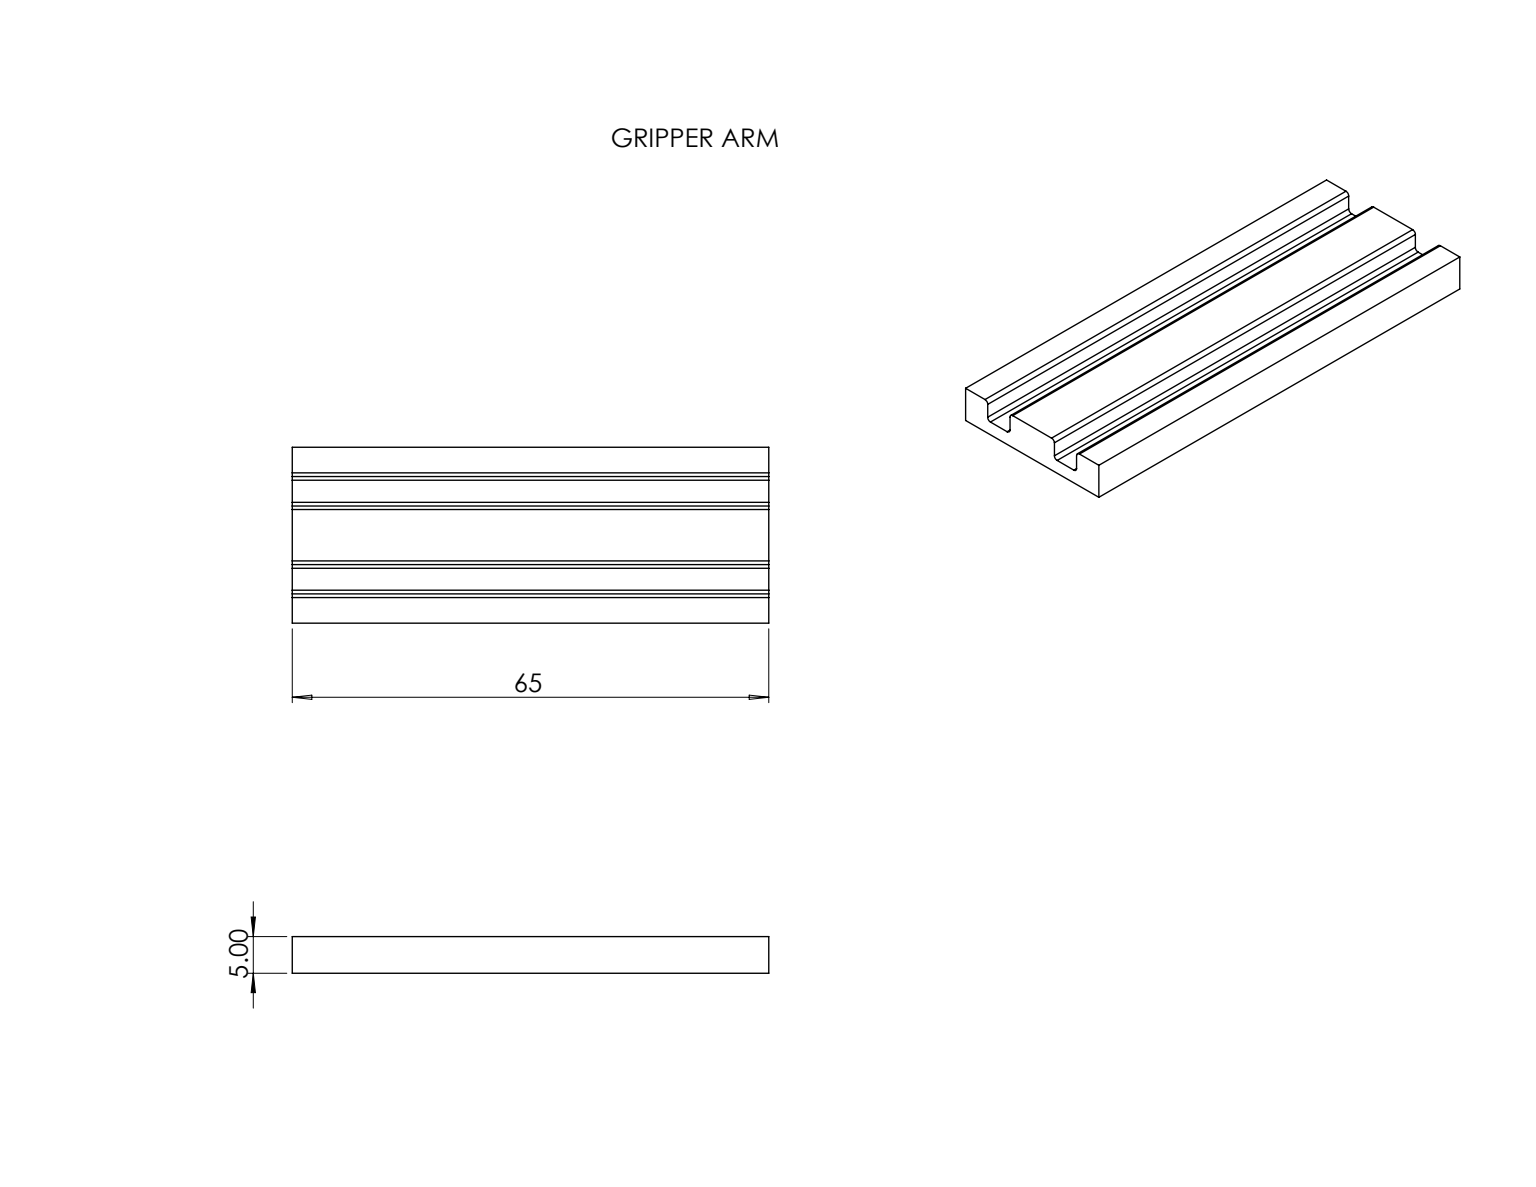
ISO-10303-21;
HEADER;
FILE_DESCRIPTION (('STEP AP214'),
    '1' );
FILE_NAME ('Gripper Arm.step',
    '2026-10-07T17:53:07',
    ( '' ),
    ( '' ),
    'SwSTEP 2.0',
    'SolidWorks 2025',
    '' );
FILE_SCHEMA (( 'AUTOMOTIVE_DESIGN' ));
ENDSEC;

DATA;
#37=( GEOMETRIC_REPRESENTATION_CONTEXT ( 3 ) GLOBAL_UNCERTAINTY_ASSIGNED_CONTEXT ( ( #1666 ) ) GLOBAL_UNIT_ASSIGNED_CONTEXT ( ( #5163, #1674, #7109 ) ) REPRESENTATION_CONTEXT ( 'NONE', 'WORKASPACE' ) );
#80=EDGE_CURVE ( 'NONE', #9144, #4985, #2152, .T. ) ;
#98=DIRECTION ( 'NONE',  ( 0.000000000000000000, 0.000000000000000000, 1.000000000000000000 ) ) ;
#126=EDGE_CURVE ( 'NONE', #1534, #5295, #6389, .T. ) ;
#133=DIRECTION ( 'NONE',  ( 0.000000000000000000, 0.000000000000000000, 1.000000000000000000 ) ) ;
#157=SHAPE_DEFINITION_REPRESENTATION ( #3699, #5502 ) ;
#159=VERTEX_POINT ( 'NONE', #3135 ) ;
#161=EDGE_CURVE ( 'NONE', #11468, #4985, #9362, .T. ) ;
#166=VECTOR ( 'NONE', #7008, 1000.000000000000000 ) ;
#169=CARTESIAN_POINT ( 'NONE',  ( 3.500000000000001776, 2.000000000000000000, 0.000000000000000000 ) ) ;
#177=VECTOR ( 'NONE', #8514, 1000.000000000000000 ) ;
#257=CYLINDRICAL_SURFACE ( 'NONE', #13000, 0.5000000000000004441 ) ;
#264=CARTESIAN_POINT ( 'NONE',  ( -3.499999999999998224, 2.499999999999999556, 0.000000000000000000 ) ) ;
#274=DIRECTION ( 'NONE',  ( 0.000000000000000000, 1.000000000000000000, 0.000000000000000000 ) ) ;
#275=FACE_OUTER_BOUND ( 'NONE', #13534, .T. ) ;
#280=VECTOR ( 'NONE', #607, 1000.000000000000000 ) ;
#294=DIRECTION ( 'NONE',  ( 0.000000000000000000, 0.000000000000000000, 1.000000000000000000 ) ) ;
#317=ORIENTED_EDGE ( 'NONE', *, *, #5380, .F. ) ;
#339=DIRECTION ( 'NONE',  ( -0.000000000000000000, -0.000000000000000000, -1.000000000000000000 ) ) ;
#366=ORIENTED_EDGE ( 'NONE', *, *, #1120, .F. ) ;
#378=LINE ( 'NONE', #13236, #10194 ) ;
#379=ORIENTED_EDGE ( 'NONE', *, *, #12753, .T. ) ;
#391=ORIENTED_EDGE ( 'NONE', *, *, #1074, .T. ) ;
#401=LINE ( 'NONE', #12069, #13543 ) ;
#408=DIRECTION ( 'NONE',  ( -1.239088197126292296E-16, 1.000000000000000000, 0.000000000000000000 ) ) ;
#414=EDGE_CURVE ( 'NONE', #159, #13667, #776, .T. ) ;
#426=CARTESIAN_POINT ( 'NONE',  ( -7.499999999999996447, -0.5000000000000019984, 0.000000000000000000 ) ) ;
#427=PLANE ( 'NONE',  #8021 ) ;
#431=ORIENTED_EDGE ( 'NONE', *, *, #1519, .T. ) ;
#490=EDGE_CURVE ( 'NONE', #10813, #8384, #10834, .T. ) ;
#544=EDGE_CURVE ( 'NONE', #2553, #8162, #1184, .T. ) ;
#571=ORIENTED_EDGE ( 'NONE', *, *, #161, .T. ) ;
#607=DIRECTION ( 'NONE',  ( -1.000000000000000000, -1.239088197126292296E-16, -0.000000000000000000 ) ) ;
#627=DIRECTION ( 'NONE',  ( -0.000000000000000000, -0.000000000000000000, -1.000000000000000000 ) ) ;
#631=ORIENTED_EDGE ( 'NONE', *, *, #12993, .T. ) ;
#646=CIRCLE ( 'NONE', #2677, 0.5000000000000004441 ) ;
#654=CARTESIAN_POINT ( 'NONE',  ( 4.500000000000002665, -0.5000000000000005551, 0.000000000000000000 ) ) ;
#657=LINE ( 'NONE', #12469, #5078 ) ;
#683=VECTOR ( 'NONE', #6615, 1000.000000000000000 ) ;
#685=ORIENTED_EDGE ( 'NONE', *, *, #926, .F. ) ;
#687=DIRECTION ( 'NONE',  ( 1.000000000000000000, 0.000000000000000000, 0.000000000000000000 ) ) ;
#694=FACE_OUTER_BOUND ( 'NONE', #1462, .T. ) ;
#736=EDGE_CURVE ( 'NONE', #4755, #1534, #2879, .T. ) ;
#748=DIRECTION ( 'NONE',  ( -0.000000000000000000, -0.000000000000000000, -1.000000000000000000 ) ) ;
#776=LINE ( 'NONE', #13553, #11837 ) ;
#789=EDGE_CURVE ( 'NONE', #2553, #2266, #4127, .T. ) ;
#797=DIRECTION ( 'NONE',  ( 0.000000000000000000, 0.000000000000000000, 1.000000000000000000 ) ) ;
#825=SURFACE_SIDE_STYLE ('',( #2881 ) ) ;
#870=CARTESIAN_POINT ( 'NONE',  ( 3.500000000000001776, 2.000000000000000000, -65.00000000000000000 ) ) ;
#886=FACE_OUTER_BOUND ( 'NONE', #3660, .T. ) ;
#891=ADVANCED_FACE ( 'NONE', ( #3224 ), #10819, .T. ) ;
#901=DIRECTION ( 'NONE',  ( 0.000000000000000000, 0.000000000000000000, 1.000000000000000000 ) ) ;
#904=EDGE_CURVE ( 'NONE', #3647, #3770, #5487, .T. ) ;
#905=AXIS2_PLACEMENT_3D ( 'NONE', #10351, #13424, #6008 ) ;
#926=EDGE_CURVE ( 'NONE', #10303, #13667, #5427, .T. ) ;
#928=EDGE_CURVE ( 'NONE', #1230, #2349, #8492, .T. ) ;
#934=ADVANCED_FACE ( 'NONE', ( #275 ), #5359, .T. ) ;
#992=CARTESIAN_POINT ( 'NONE',  ( -7.499999999999996447, -1.762812401309176307E-15, -65.00000000000000000 ) ) ;
#1016=DIRECTION ( 'NONE',  ( 1.000000000000000000, 0.000000000000000000, 0.000000000000000000 ) ) ;
#1074=EDGE_CURVE ( 'NONE', #2266, #4291, #7792, .T. ) ;
#1075=( GEOMETRIC_REPRESENTATION_CONTEXT ( 3 ) GLOBAL_UNCERTAINTY_ASSIGNED_CONTEXT ( ( #1813 ) ) GLOBAL_UNIT_ASSIGNED_CONTEXT ( ( #10879, #7487, #2162 ) ) REPRESENTATION_CONTEXT ( 'NONE', 'WORKASPACE' ) );
#1077=ORIENTED_EDGE ( 'NONE', *, *, #9933, .F. ) ;
#1098=DIRECTION ( 'NONE',  ( -1.000000000000000000, 5.059610138265691632E-16, 0.000000000000000000 ) ) ;
#1120=EDGE_CURVE ( 'NONE', #8521, #2257, #4929, .T. ) ;
#1162=ORIENTED_EDGE ( 'NONE', *, *, #6210, .T. ) ;
#1167=EDGE_CURVE ( 'NONE', #10572, #8384, #2508, .T. ) ;
#1184=LINE ( 'NONE', #9716, #3596 ) ;
#1192=LINE ( 'NONE', #12999, #11798 ) ;
#1196=ORIENTED_EDGE ( 'NONE', *, *, #10990, .T. ) ;
#1222=CARTESIAN_POINT ( 'NONE',  ( -8.500000000000000000, 2.499999999999999556, -65.00000000000000000 ) ) ;
#1230=VERTEX_POINT ( 'NONE', #9272 ) ;
#1245=ORIENTED_EDGE ( 'NONE', *, *, #8673, .T. ) ;
#1246=VECTOR ( 'NONE', #11216, 1000.000000000000000 ) ;
#1258=ORIENTED_EDGE ( 'NONE', *, *, #10990, .F. ) ;
#1259=ORIENTED_EDGE ( 'NONE', *, *, #7216, .F. ) ;
#1303=FACE_OUTER_BOUND ( 'NONE', #3883, .T. ) ;
#1373=CARTESIAN_POINT ( 'NONE',  ( 3.500000000000001776, 2.499999999999999556, 0.000000000000000000 ) ) ;
#1380=DIRECTION ( 'NONE',  ( -1.000000000000000000, -2.529805069132845816E-16, 0.000000000000000000 ) ) ;
#1385=CARTESIAN_POINT ( 'NONE',  ( 7.500000000000000000, -0.5000000000000017764, -65.00000000000000000 ) ) ;
#1407=EDGE_CURVE ( 'NONE', #8384, #9884, #13503, .T. ) ;
#1437=PLANE ( 'NONE',  #8954 ) ;
#1462=EDGE_LOOP ( 'NONE', ( #7418, #7086, #12382, #7454 ) ) ;
#1476=ORIENTED_EDGE ( 'NONE', *, *, #13544, .T. ) ;
#1493=EDGE_LOOP ( 'NONE', ( #9757, #11508, #6256, #13606 ) ) ;
#1519=EDGE_CURVE ( 'NONE', #5154, #11963, #6379, .T. ) ;
#1534=VERTEX_POINT ( 'NONE', #11903 ) ;
#1608=COLOUR_RGB ( '', 0.08235294, 0.09019608, 0.10196078) ;
#1613=DIRECTION ( 'NONE',  ( 1.000000000000000000, 0.000000000000000000, -0.000000000000000000 ) ) ;
#1620=ORIENTED_EDGE ( 'NONE', *, *, #9892, .T. ) ;
#1648=EDGE_CURVE ( 'NONE', #4985, #10572, #10929, .T. ) ;
#1649=EDGE_LOOP ( 'NONE', ( #12050, #2259, #5190, #4837 ) ) ;
#1658=ORIENTED_EDGE ( 'NONE', *, *, #1074, .F. ) ;
#1660=LINE ( 'NONE', #7289, #5099 ) ;
#1666=UNCERTAINTY_MEASURE_WITH_UNIT (LENGTH_MEASURE( 1.000000000000000082E-05 ), #5163, 'distance_accuracy_value', 'NONE');
#1671=ORIENTED_EDGE ( 'NONE', *, *, #1519, .F. ) ;
#1674=( NAMED_UNIT ( * ) PLANE_ANGLE_UNIT ( ) SI_UNIT ( $, .RADIAN. ) );
#1706=DIRECTION ( 'NONE',  ( 0.000000000000000000, 0.000000000000000000, 1.000000000000000000 ) ) ;
#1719=ORIENTED_EDGE ( 'NONE', *, *, #11656, .T. ) ;
#1745=AXIS2_PLACEMENT_3D ( 'NONE', #12207, #274, #3424 ) ;
#1764=CARTESIAN_POINT ( 'NONE',  ( 12.00000000000000000, -2.499999999999999556, -65.00000000000000000 ) ) ;
#1796=CARTESIAN_POINT ( 'NONE',  ( 7.500000000000000000, -0.5000000000000017764, 0.000000000000000000 ) ) ;
#1813=UNCERTAINTY_MEASURE_WITH_UNIT (LENGTH_MEASURE( 1.000000000000000082E-05 ), #10879, 'distance_accuracy_value', 'NONE');
#1815=AXIS2_PLACEMENT_3D ( 'NONE', #2245, #11724, #9640 ) ;
#1823=DIRECTION ( 'NONE',  ( 0.000000000000000000, 0.000000000000000000, 1.000000000000000000 ) ) ;
#1859=CARTESIAN_POINT ( 'NONE',  ( -4.499999999999999112, -1.301042606982605321E-15, -65.00000000000000000 ) ) ;
#1900=ORIENTED_EDGE ( 'NONE', *, *, #12612, .F. ) ;
#1914=ORIENTED_EDGE ( 'NONE', *, *, #5344, .T. ) ;
#1917=EDGE_CURVE ( 'NONE', #3017, #10813, #3374, .T. ) ;
#1919=AXIS2_PLACEMENT_3D ( 'NONE', #10965, #5557, #1380 ) ;
#1940=LINE ( 'NONE', #6111, #280 ) ;
#1965=ADVANCED_FACE ( 'NONE', ( #10130 ), #10060, .T. ) ;
#1983=DIRECTION ( 'NONE',  ( 0.000000000000000000, 0.000000000000000000, 1.000000000000000000 ) ) ;
#1992=VECTOR ( 'NONE', #10685, 1000.000000000000000 ) ;
#1999=ORIENTED_EDGE ( 'NONE', *, *, #9250, .F. ) ;
#2000=AXIS2_PLACEMENT_3D ( 'NONE', #6057, #11507, #10460 ) ;
#2018=AXIS2_PLACEMENT_3D ( 'NONE', #10654, #10728, #1016 ) ;
#2048=VECTOR ( 'NONE', #8009, 1000.000000000000000 ) ;
#2065=VECTOR ( 'NONE', #4779, 1000.000000000000000 ) ;
#2114=ADVANCED_FACE ( 'NONE', ( #886 ), #7167, .T. ) ;
#2151=CARTESIAN_POINT ( 'NONE',  ( 4.500000000000002665, -0.5000000000000005551, -65.00000000000000000 ) ) ;
#2152=LINE ( 'NONE', #12953, #13752 ) ;
#2153=LINE ( 'NONE', #4239, #9391 ) ;
#2160=DIRECTION ( 'NONE',  ( 0.000000000000000000, 1.000000000000000000, 0.000000000000000000 ) ) ;
#2162=( NAMED_UNIT ( * ) SI_UNIT ( $, .STERADIAN. ) SOLID_ANGLE_UNIT ( ) );
#2168=ORIENTED_EDGE ( 'NONE', *, *, #126, .T. ) ;
#2172=DIRECTION ( 'NONE',  ( 1.000000000000000000, 0.000000000000000000, 0.000000000000000000 ) ) ;
#2205=CARTESIAN_POINT ( 'NONE',  ( 8.500000000000003553, 2.500000000000000000, 0.000000000000000000 ) ) ;
#2239=ORIENTED_EDGE ( 'NONE', *, *, #7229, .F. ) ;
#2245=CARTESIAN_POINT ( 'NONE',  ( 8.500000000000001776, 2.000000000000000000, -65.00000000000000000 ) ) ;
#2257=VERTEX_POINT ( 'NONE', #10663 ) ;
#2259=ORIENTED_EDGE ( 'NONE', *, *, #544, .F. ) ;
#2266=VERTEX_POINT ( 'NONE', #6674 ) ;
#2306=EDGE_CURVE ( 'NONE', #4291, #159, #7705, .T. ) ;
#2347=VERTEX_POINT ( 'NONE', #1373 ) ;
#2349=VERTEX_POINT ( 'NONE', #1222 ) ;
#2367=VERTEX_POINT ( 'NONE', #7563 ) ;
#2380=VERTEX_POINT ( 'NONE', #4381 ) ;
#2389=CARTESIAN_POINT ( 'NONE',  ( -3.499999999999998224, 2.499999999999999556, -65.00000000000000000 ) ) ;
#2409=ADVANCED_FACE ( 'NONE', ( #5828 ), #1437, .T. ) ;
#2462=VECTOR ( 'NONE', #11651, 1000.000000000000000 ) ;
#2466=LINE ( 'NONE', #9005, #10134 ) ;
#2497=DIRECTION ( 'NONE',  ( -0.000000000000000000, 1.000000000000000000, -0.000000000000000000 ) ) ;
#2508=CIRCLE ( 'NONE', #6274, 0.5000000000000004441 ) ;
#2511=CARTESIAN_POINT ( 'NONE',  ( -7.999999999999996447, -1.701580061351808733E-15, -65.00000000000000000 ) ) ;
#2540=ORIENTED_EDGE ( 'NONE', *, *, #4860, .F. ) ;
#2553=VERTEX_POINT ( 'NONE', #11356 ) ;
#2677=AXIS2_PLACEMENT_3D ( 'NONE', #10326, #748, #9275 ) ;
#2689=VECTOR ( 'NONE', #6333, 1000.000000000000000 ) ;
#2717=LINE ( 'NONE', #11284, #6753 ) ;
#2718=LINE ( 'NONE', #7210, #166 ) ;
#2741=CARTESIAN_POINT ( 'NONE',  ( 12.00000000000000000, 2.500000000000000000, 0.000000000000000000 ) ) ;
#2848=ORIENTED_EDGE ( 'NONE', *, *, #6277, .F. ) ;
#2852=DIRECTION ( 'NONE',  ( 0.000000000000000000, 0.000000000000000000, 1.000000000000000000 ) ) ;
#2854=DIRECTION ( 'NONE',  ( 0.000000000000000000, 0.000000000000000000, 1.000000000000000000 ) ) ;
#2879=LINE ( 'NONE', #13538, #11401 ) ;
#2881=SURFACE_STYLE_FILL_AREA ( #13409 ) ;
#2904=CYLINDRICAL_SURFACE ( 'NONE', #9563, 0.5000000000000004441 ) ;
#2965=EDGE_CURVE ( 'NONE', #13584, #12422, #13356, .T. ) ;
#2983=CARTESIAN_POINT ( 'NONE',  ( 8.000000000000000000, -1.762812401309176307E-15, -65.00000000000000000 ) ) ;
#3017=VERTEX_POINT ( 'NONE', #2983 ) ;
#3031=CYLINDRICAL_SURFACE ( 'NONE', #5960, 0.4999999999999991673 ) ;
#3071=CARTESIAN_POINT ( 'NONE',  ( 7.500000000000000000, -1.762812401309176307E-15, 0.000000000000000000 ) ) ;
#3082=FACE_OUTER_BOUND ( 'NONE', #12101, .T. ) ;
#3085=CARTESIAN_POINT ( 'NONE',  ( -12.00000000000000000, -2.500000000000000444, -65.00000000000000000 ) ) ;
#3099=CIRCLE ( 'NONE', #8884, 0.4999999999999991673 ) ;
#3131=EDGE_CURVE ( 'NONE', #11544, #11152, #4409, .T. ) ;
#3135=CARTESIAN_POINT ( 'NONE',  ( 12.00000000000000000, 2.500000000000000000, -65.00000000000000000 ) ) ;
#3142=CARTESIAN_POINT ( 'NONE',  ( 4.000000000000001776, 2.000000000000000000, -65.00000000000000000 ) ) ;
#3216=ORIENTED_EDGE ( 'NONE', *, *, #6210, .F. ) ;
#3224=FACE_OUTER_BOUND ( 'NONE', #4359, .T. ) ;
#3259=ADVANCED_FACE ( 'NONE', ( #6715 ), #427, .T. ) ;
#3263=ADVANCED_FACE ( 'NONE', ( #6840 ), #9932, .T. ) ;
#3276=CARTESIAN_POINT ( 'NONE',  ( -12.00000000000000000, 2.500000000000000000, 0.000000000000000000 ) ) ;
#3336=DIRECTION ( 'NONE',  ( 0.000000000000000000, -1.000000000000000000, 0.000000000000000000 ) ) ;
#3343=EDGE_LOOP ( 'NONE', ( #5355, #571, #8847, #13069, #9284, #8231, #13676, #5582, #12581, #8099, #2168, #9530, #11277, #5885, #6832, #13165, #1162, #8173, #631, #10642 ) ) ;
#3344=ORIENTED_EDGE ( 'NONE', *, *, #8167, .F. ) ;
#3350=VECTOR ( 'NONE', #13795, 1000.000000000000000 ) ;
#3374=CIRCLE ( 'NONE', #10066, 0.5000000000000004441 ) ;
#3407=DIRECTION ( 'NONE',  ( 0.000000000000000000, 0.000000000000000000, 1.000000000000000000 ) ) ;
#3412=CARTESIAN_POINT ( 'NONE',  ( 12.00000000000000000, -2.499999999999999556, -65.00000000000000000 ) ) ;
#3417=ORIENTED_EDGE ( 'NONE', *, *, #904, .F. ) ;
#3424=DIRECTION ( 'NONE',  ( 0.000000000000000000, -0.000000000000000000, 1.000000000000000000 ) ) ;
#3455=EDGE_CURVE ( 'NONE', #11963, #3647, #4031, .T. ) ;
#3464=ORIENTED_EDGE ( 'NONE', *, *, #12753, .F. ) ;
#3488=DIRECTION ( 'NONE',  ( -1.000000000000000000, 0.000000000000000000, 0.000000000000000000 ) ) ;
#3516=ORIENTED_EDGE ( 'NONE', *, *, #12993, .F. ) ;
#3517=VECTOR ( 'NONE', #7581, 1000.000000000000000 ) ;
#3559=CARTESIAN_POINT ( 'NONE',  ( -12.00000000000000000, -2.500000000000000444, 0.000000000000000000 ) ) ;
#3588=ORIENTED_EDGE ( 'NONE', *, *, #8167, .T. ) ;
#3591=ORIENTED_EDGE ( 'NONE', *, *, #1120, .T. ) ;
#3592=EDGE_CURVE ( 'NONE', #3770, #4357, #4258, .T. ) ;
#3596=VECTOR ( 'NONE', #4403, 1000.000000000000000 ) ;
#3612=CARTESIAN_POINT ( 'NONE',  ( 8.000000000000001776, 2.000000000000000000, -65.00000000000000000 ) ) ;
#3627=VERTEX_POINT ( 'NONE', #3559 ) ;
#3647=VERTEX_POINT ( 'NONE', #12974 ) ;
#3660=EDGE_LOOP ( 'NONE', ( #9021, #12465, #5916, #10909 ) ) ;
#3664=CARTESIAN_POINT ( 'NONE',  ( 3.500000000000001776, 2.499999999999999556, -65.00000000000000000 ) ) ;
#3687=CARTESIAN_POINT ( 'NONE',  ( -8.499999999999998224, 2.000000000000000000, 0.000000000000000000 ) ) ;
#3697=CARTESIAN_POINT ( 'NONE',  ( -12.00000000000000000, -2.500000000000000444, -65.00000000000000000 ) ) ;
#3699=PRODUCT_DEFINITION_SHAPE ( 'NONE', 'NONE',  #10061 ) ;
#3744=PLANE ( 'NONE',  #4196 ) ;
#3753=CARTESIAN_POINT ( 'NONE',  ( -12.00000000000000000, 2.500000000000000000, 0.000000000000000000 ) ) ;
#3754=DIRECTION ( 'NONE',  ( 1.000000000000000000, 0.000000000000000000, 0.000000000000000000 ) ) ;
#3770=VERTEX_POINT ( 'NONE', #6047 ) ;
#3843=DIRECTION ( 'NONE',  ( -1.000000000000000000, 0.000000000000000000, 0.000000000000000000 ) ) ;
#3883=EDGE_LOOP ( 'NONE', ( #10092, #9235, #13516, #431 ) ) ;
#3888=CYLINDRICAL_SURFACE ( 'NONE', #9321, 0.5000000000000004441 ) ;
#3948=EDGE_CURVE ( 'NONE', #6401, #1534, #10955, .T. ) ;
#3970=EDGE_CURVE ( 'NONE', #8162, #3627, #2153, .T. ) ;
#3977=DIRECTION ( 'NONE',  ( 1.000000000000000000, 8.673617379884027583E-16, -0.000000000000000000 ) ) ;
#3998=VERTEX_POINT ( 'NONE', #10589 ) ;
#4031=CIRCLE ( 'NONE', #10940, 0.5000000000000004441 ) ;
#4080=CARTESIAN_POINT ( 'NONE',  ( -12.00000000000000000, 2.500000000000000000, -65.00000000000000000 ) ) ;
#4082=ORIENTED_EDGE ( 'NONE', *, *, #13544, .F. ) ;
#4088=ORIENTED_EDGE ( 'NONE', *, *, #6277, .T. ) ;
#4103=ORIENTED_EDGE ( 'NONE', *, *, #126, .F. ) ;
#4127=LINE ( 'NONE', #3085, #5364 ) ;
#4188=EDGE_LOOP ( 'NONE', ( #7507, #12754, #7359, #1914 ) ) ;
#4196=AXIS2_PLACEMENT_3D ( 'NONE', #7994, #6032, #8071 ) ;
#4239=CARTESIAN_POINT ( 'NONE',  ( -12.00000000000000000, -2.500000000000000444, 0.000000000000000000 ) ) ;
#4258=CIRCLE ( 'NONE', #13615, 0.5000000000000004441 ) ;
#4273=AXIS2_PLACEMENT_3D ( 'NONE', #10752, #8789, #2172 ) ;
#4284=CARTESIAN_POINT ( 'NONE',  ( 7.500000000000000000, -0.5000000000000017764, -65.00000000000000000 ) ) ;
#4289=VECTOR ( 'NONE', #4600, 1000.000000000000000 ) ;
#4291=VERTEX_POINT ( 'NONE', #1764 ) ;
#4301=AXIS2_PLACEMENT_3D ( 'NONE', #13028, #8910, #12053 ) ;
#4308=ADVANCED_FACE ( 'NONE', ( #4909 ), #9170, .T. ) ;
#4349=LINE ( 'NONE', #4284, #12699 ) ;
#4357=VERTEX_POINT ( 'NONE', #8454 ) ;
#4359=EDGE_LOOP ( 'NONE', ( #11012, #3344, #9662, #9926 ) ) ;
#4381=CARTESIAN_POINT ( 'NONE',  ( 4.000000000000001776, 2.000000000000000000, -65.00000000000000000 ) ) ;
#4403=DIRECTION ( 'NONE',  ( 0.000000000000000000, 0.000000000000000000, 1.000000000000000000 ) ) ;
#4409=LINE ( 'NONE', #10699, #5553 ) ;
#4446=DIRECTION ( 'NONE',  ( 1.000000000000000000, 0.000000000000000000, 0.000000000000000000 ) ) ;
#4537=FACE_OUTER_BOUND ( 'NONE', #9878, .T. ) ;
#4538=CARTESIAN_POINT ( 'NONE',  ( -7.999999999999998224, 2.000000000000000000, 0.000000000000000000 ) ) ;
#4554=DIRECTION ( 'NONE',  ( -0.000000000000000000, 0.000000000000000000, -1.000000000000000000 ) ) ;
#4556=CARTESIAN_POINT ( 'NONE',  ( -12.00000000000000000, -2.500000000000000444, -65.00000000000000000 ) ) ;
#4577=MANIFOLD_SOLID_BREP ( 'Boss-Extrude1', #5904 ) ;
#4600=DIRECTION ( 'NONE',  ( 0.000000000000000000, 0.000000000000000000, 1.000000000000000000 ) ) ;
#4658=DIRECTION ( 'NONE',  ( 1.000000000000000000, 3.614007241618347908E-17, 0.000000000000000000 ) ) ;
#4672=DIRECTION ( 'NONE',  ( -1.000000000000000000, -0.000000000000000000, -0.000000000000000000 ) ) ;
#4673=PLANE ( 'NONE',  #5961 ) ;
#4686=ORIENTED_EDGE ( 'NONE', *, *, #3131, .F. ) ;
#4697=DIRECTION ( 'NONE',  ( 0.000000000000000000, 0.000000000000000000, 1.000000000000000000 ) ) ;
#4723=PLANE ( 'NONE',  #6385 ) ;
#4755=VERTEX_POINT ( 'NONE', #8931 ) ;
#4762=DIRECTION ( 'NONE',  ( 1.000000000000000000, 0.000000000000000000, -0.000000000000000000 ) ) ;
#4779=DIRECTION ( 'NONE',  ( -8.673617379884027583E-16, -1.000000000000000000, 0.000000000000000000 ) ) ;
#4801=CARTESIAN_POINT ( 'NONE',  ( -3.999999999999997335, 2.000000000000000000, -65.00000000000000000 ) ) ;
#4814=EDGE_CURVE ( 'NONE', #1230, #3770, #13047, .T. ) ;
#4837=ORIENTED_EDGE ( 'NONE', *, *, #7216, .T. ) ;
#4860=EDGE_CURVE ( 'NONE', #159, #3998, #1940, .T. ) ;
#4909=FACE_OUTER_BOUND ( 'NONE', #10314, .T. ) ;
#4919=AXIS2_PLACEMENT_3D ( 'NONE', #11709, #9684, #9611 ) ;
#4925=DIRECTION ( 'NONE',  ( -1.000000000000000000, -2.529805069132845816E-16, -0.000000000000000000 ) ) ;
#4929=CIRCLE ( 'NONE', #12736, 0.5000000000000004441 ) ;
#4944=CARTESIAN_POINT ( 'NONE',  ( 8.000000000000001776, 2.000000000000000000, 0.000000000000000000 ) ) ;
#4956=PLANE ( 'NONE',  #8585 ) ;
#4985=VERTEX_POINT ( 'NONE', #4944 ) ;
#4990=DIRECTION ( 'NONE',  ( -1.000000000000000000, 0.000000000000000000, 0.000000000000000000 ) ) ;
#5078=VECTOR ( 'NONE', #4925, 1000.000000000000000 ) ;
#5079=CIRCLE ( 'NONE', #6862, 0.5000000000000004441 ) ;
#5099=VECTOR ( 'NONE', #8088, 1000.000000000000000 ) ;
#5107=DIRECTION ( 'NONE',  ( 0.000000000000000000, 0.000000000000000000, 1.000000000000000000 ) ) ;
#5154=VERTEX_POINT ( 'NONE', #9833 ) ;
#5163=( LENGTH_UNIT ( ) NAMED_UNIT ( * ) SI_UNIT ( .MILLI., .METRE. ) );
#5181=EDGE_CURVE ( 'NONE', #8888, #2367, #12766, .T. ) ;
#5186=EDGE_CURVE ( 'NONE', #13667, #11468, #13095, .T. ) ;
#5190=ORIENTED_EDGE ( 'NONE', *, *, #789, .T. ) ;
#5204=ORIENTED_EDGE ( 'NONE', *, *, #789, .F. ) ;
#5229=ADVANCED_FACE ( 'NONE', ( #8834 ), #257, .F. ) ;
#5290=CARTESIAN_POINT ( 'NONE',  ( -3.999999999999998224, -1.301042606982605321E-15, -65.00000000000000000 ) ) ;
#5295=VERTEX_POINT ( 'NONE', #5824 ) ;
#5302=CARTESIAN_POINT ( 'NONE',  ( -3.999999999999998224, -1.301042606982605321E-15, -65.00000000000000000 ) ) ;
#5321=VECTOR ( 'NONE', #6748, 1000.000000000000000 ) ;
#5324=DIRECTION ( 'NONE',  ( 0.000000000000000000, 0.000000000000000000, 1.000000000000000000 ) ) ;
#5344=EDGE_CURVE ( 'NONE', #3017, #10572, #2717, .T. ) ;
#5355=ORIENTED_EDGE ( 'NONE', *, *, #5186, .T. ) ;
#5359=PLANE ( 'NONE',  #12063 ) ;
#5364=VECTOR ( 'NONE', #12574, 1000.000000000000000 ) ;
#5380=EDGE_CURVE ( 'NONE', #3998, #9144, #9659, .T. ) ;
#5381=STYLED_ITEM ( 'NONE', ( #5994 ), #4577 ) ;
#5384=ORIENTED_EDGE ( 'NONE', *, *, #11656, .F. ) ;
#5400=PRODUCT ( 'Gripper Arm', 'Gripper Arm', '', ( #9120 ) ) ;
#5406=CARTESIAN_POINT ( 'NONE',  ( -3.999999999999997335, 2.000000000000000000, 0.000000000000000000 ) ) ;
#5411=EDGE_LOOP ( 'NONE', ( #9740, #6725, #379, #6459 ) ) ;
#5412=CARTESIAN_POINT ( 'NONE',  ( 7.500000000000000000, -0.5000000000000017764, -65.00000000000000000 ) ) ;
#5427=LINE ( 'NONE', #10679, #12947 ) ;
#5449=EDGE_LOOP ( 'NONE', ( #11527, #8507, #9407, #3588 ) ) ;
#5487=LINE ( 'NONE', #4538, #683 ) ;
#5502=SHAPE_REPRESENTATION ( 'Gripper Arm', ( #6434 ), #1075 ) ;
#5553=VECTOR ( 'NONE', #8591, 1000.000000000000000 ) ;
#5557=DIRECTION ( 'NONE',  ( -2.529805069132845816E-16, 1.000000000000000000, 0.000000000000000000 ) ) ;
#5563=PLANE ( 'NONE',  #12226 ) ;
#5582=ORIENTED_EDGE ( 'NONE', *, *, #9638, .T. ) ;
#5635=FACE_OUTER_BOUND ( 'NONE', #9619, .T. ) ;
#5642=PLANE ( 'NONE',  #9345 ) ;
#5742=DIRECTION ( 'NONE',  ( 0.000000000000000000, 0.000000000000000000, 1.000000000000000000 ) ) ;
#5758=CIRCLE ( 'NONE', #2000, 0.5000000000000004441 ) ;
#5768=PLANE ( 'NONE',  #1745 ) ;
#5824=CARTESIAN_POINT ( 'NONE',  ( -3.999999999999998224, -1.301042606982605321E-15, 0.000000000000000000 ) ) ;
#5828=FACE_OUTER_BOUND ( 'NONE', #10292, .T. ) ;
#5836=DIRECTION ( 'NONE',  ( 0.000000000000000000, 0.000000000000000000, 1.000000000000000000 ) ) ;
#5848=CARTESIAN_POINT ( 'NONE',  ( 4.000000000000001776, -4.336808689942017736E-16, 0.000000000000000000 ) ) ;
#5870=ORIENTED_EDGE ( 'NONE', *, *, #12293, .F. ) ;
#5871=ORIENTED_EDGE ( 'NONE', *, *, #5181, .F. ) ;
#5885=ORIENTED_EDGE ( 'NONE', *, *, #3455, .T. ) ;
#5887=EDGE_CURVE ( 'NONE', #2257, #13584, #2466, .T. ) ;
#5888=LINE ( 'NONE', #12585, #1246 ) ;
#5904=CLOSED_SHELL ( 'NONE', ( #1965, #11164, #2409, #13657, #4308, #13050, #7932, #11655, #8241, #5229, #11071, #13376, #11086, #2114, #3263, #9132, #934, #6518, #8578, #891, #13014, #3259 ) ) ;
#5916=ORIENTED_EDGE ( 'NONE', *, *, #6474, .T. ) ;
#5940=ORIENTED_EDGE ( 'NONE', *, *, #1407, .F. ) ;
#5960=AXIS2_PLACEMENT_3D ( 'NONE', #7242, #11521, #8380 ) ;
#5961=AXIS2_PLACEMENT_3D ( 'NONE', #4801, #3488, #12978 ) ;
#5994=PRESENTATION_STYLE_ASSIGNMENT (( #11255 ) ) ;
#6008=DIRECTION ( 'NONE',  ( -1.000000000000000000, 1.239088197126291063E-16, 0.000000000000000000 ) ) ;
#6009=ORIENTED_EDGE ( 'NONE', *, *, #8562, .T. ) ;
#6032=DIRECTION ( 'NONE',  ( 0.000000000000000000, 0.000000000000000000, 1.000000000000000000 ) ) ;
#6047=CARTESIAN_POINT ( 'NONE',  ( -7.999999999999998224, 2.000000000000000000, 0.000000000000000000 ) ) ;
#6057=CARTESIAN_POINT ( 'NONE',  ( 4.500000000000002665, -4.336808689942017736E-16, 0.000000000000000000 ) ) ;
#6078=LINE ( 'NONE', #4080, #8652 ) ;
#6110=DIRECTION ( 'NONE',  ( -0.000000000000000000, -0.000000000000000000, -1.000000000000000000 ) ) ;
#6111=CARTESIAN_POINT ( 'NONE',  ( 8.500000000000003553, 2.499999999999999556, -65.00000000000000000 ) ) ;
#6157=ORIENTED_EDGE ( 'NONE', *, *, #736, .F. ) ;
#6199=FILL_AREA_STYLE_COLOUR ( '', #1608 ) ;
#6208=VECTOR ( 'NONE', #12193, 1000.000000000000000 ) ;
#6210=EDGE_CURVE ( 'NONE', #4357, #8162, #8561, .T. ) ;
#6256=ORIENTED_EDGE ( 'NONE', *, *, #928, .T. ) ;
#6274=AXIS2_PLACEMENT_3D ( 'NONE', #3071, #6110, #7355 ) ;
#6277=EDGE_CURVE ( 'NONE', #4755, #8888, #6543, .T. ) ;
#6281=CARTESIAN_POINT ( 'NONE',  ( 4.500000000000002665, -4.336808689942017736E-16, -65.00000000000000000 ) ) ;
#6333=DIRECTION ( 'NONE',  ( 0.000000000000000000, -1.000000000000000000, 0.000000000000000000 ) ) ;
#6353=EDGE_LOOP ( 'NONE', ( #11064, #1671, #12134, #1196 ) ) ;
#6379=LINE ( 'NONE', #8681, #7367 ) ;
#6385=AXIS2_PLACEMENT_3D ( 'NONE', #3612, #13089, #11913 ) ;
#6389=LINE ( 'NONE', #5406, #2689 ) ;
#6394=ORIENTED_EDGE ( 'NONE', *, *, #1917, .F. ) ;
#6401=VERTEX_POINT ( 'NONE', #264 ) ;
#6411=LINE ( 'NONE', #5290, #1992 ) ;
#6423=ORIENTED_EDGE ( 'NONE', *, *, #2306, .T. ) ;
#6434=AXIS2_PLACEMENT_3D ( 'NONE', #11654, #12825, #11856 ) ;
#6444=ORIENTED_EDGE ( 'NONE', *, *, #928, .F. ) ;
#6459=ORIENTED_EDGE ( 'NONE', *, *, #12551, .T. ) ;
#6474=EDGE_CURVE ( 'NONE', #2380, #11544, #9822, .T. ) ;
#6499=ORIENTED_EDGE ( 'NONE', *, *, #5181, .T. ) ;
#6518=ADVANCED_FACE ( 'NONE', ( #11222 ), #6950, .F. ) ;
#6524=DIRECTION ( 'NONE',  ( 1.000000000000000000, 0.000000000000000000, 0.000000000000000000 ) ) ;
#6543=LINE ( 'NONE', #9692, #7331 ) ;
#6602=VECTOR ( 'NONE', #10651, 1000.000000000000000 ) ;
#6615=DIRECTION ( 'NONE',  ( -8.673617379884027583E-16, 1.000000000000000000, -0.000000000000000000 ) ) ;
#6618=DIRECTION ( 'NONE',  ( -0.000000000000000000, -0.000000000000000000, -1.000000000000000000 ) ) ;
#6674=CARTESIAN_POINT ( 'NONE',  ( -12.00000000000000000, -2.500000000000000444, -65.00000000000000000 ) ) ;
#6715=FACE_OUTER_BOUND ( 'NONE', #3343, .T. ) ;
#6725=ORIENTED_EDGE ( 'NONE', *, *, #5887, .F. ) ;
#6748=DIRECTION ( 'NONE',  ( 0.000000000000000000, 0.000000000000000000, 1.000000000000000000 ) ) ;
#6753=VECTOR ( 'NONE', #1706, 1000.000000000000000 ) ;
#6760=DIRECTION ( 'NONE',  ( 0.000000000000000000, 0.000000000000000000, -1.000000000000000000 ) ) ;
#6768=DIRECTION ( 'NONE',  ( 0.000000000000000000, 0.000000000000000000, 1.000000000000000000 ) ) ;
#6811=ORIENTED_EDGE ( 'NONE', *, *, #414, .T. ) ;
#6815=CARTESIAN_POINT ( 'NONE',  ( 8.500000000000003553, 2.500000000000000000, -65.00000000000000000 ) ) ;
#6832=ORIENTED_EDGE ( 'NONE', *, *, #904, .T. ) ;
#6840=FACE_OUTER_BOUND ( 'NONE', #5411, .T. ) ;
#6862=AXIS2_PLACEMENT_3D ( 'NONE', #10852, #11826, #8604 ) ;
#6936=VECTOR ( 'NONE', #2160, 1000.000000000000000 ) ;
#6950=CYLINDRICAL_SURFACE ( 'NONE', #10269, 0.5000000000000004441 ) ;
#6964=VECTOR ( 'NONE', #7702, 1000.000000000000000 ) ;
#7008=DIRECTION ( 'NONE',  ( 1.000000000000000000, 3.614007241618347908E-17, 0.000000000000000000 ) ) ;
#7009=CARTESIAN_POINT ( 'NONE',  ( -12.00000000000000000, -2.500000000000000444, -65.00000000000000000 ) ) ;
#7086=ORIENTED_EDGE ( 'NONE', *, *, #8673, .F. ) ;
#7088=DIRECTION ( 'NONE',  ( -8.673617379884027583E-16, 1.000000000000000000, -0.000000000000000000 ) ) ;
#7109=( NAMED_UNIT ( * ) SI_UNIT ( $, .STERADIAN. ) SOLID_ANGLE_UNIT ( ) );
#7138=VECTOR ( 'NONE', #133, 1000.000000000000000 ) ;
#7145=CARTESIAN_POINT ( 'NONE',  ( -4.499999999999999112, -0.5000000000000009992, -65.00000000000000000 ) ) ;
#7167=CYLINDRICAL_SURFACE ( 'NONE', #8044, 0.5000000000000000000 ) ;
#7172=ORIENTED_EDGE ( 'NONE', *, *, #8767, .F. ) ;
#7210=CARTESIAN_POINT ( 'NONE',  ( -12.00000000000000000, -2.500000000000000444, 0.000000000000000000 ) ) ;
#7212=DIRECTION ( 'NONE',  ( 1.000000000000000000, 0.000000000000000000, 0.000000000000000000 ) ) ;
#7216=EDGE_CURVE ( 'NONE', #2266, #3627, #12095, .T. ) ;
#7229=EDGE_CURVE ( 'NONE', #9144, #3017, #1192, .T. ) ;
#7242=CARTESIAN_POINT ( 'NONE',  ( -3.499999999999998224, 2.000000000000000000, -65.00000000000000000 ) ) ;
#7289=CARTESIAN_POINT ( 'NONE',  ( 4.000000000000001776, 2.000000000000000000, -65.00000000000000000 ) ) ;
#7298=DIRECTION ( 'NONE',  ( -8.673617379884027583E-16, 1.000000000000000000, 0.000000000000000000 ) ) ;
#7331=VECTOR ( 'NONE', #3336, 1000.000000000000000 ) ;
#7355=DIRECTION ( 'NONE',  ( 1.000000000000000000, 0.000000000000000000, 0.000000000000000000 ) ) ;
#7359=ORIENTED_EDGE ( 'NONE', *, *, #7229, .T. ) ;
#7367=VECTOR ( 'NONE', #13770, 1000.000000000000000 ) ;
#7396=AXIS2_PLACEMENT_3D ( 'NONE', #10644, #5324, #8472 ) ;
#7418=ORIENTED_EDGE ( 'NONE', *, *, #3948, .F. ) ;
#7439=LINE ( 'NONE', #10613, #177 ) ;
#7454=ORIENTED_EDGE ( 'NONE', *, *, #736, .T. ) ;
#7487=( NAMED_UNIT ( * ) PLANE_ANGLE_UNIT ( ) SI_UNIT ( $, .RADIAN. ) );
#7507=ORIENTED_EDGE ( 'NONE', *, *, #1648, .F. ) ;
#7563=CARTESIAN_POINT ( 'NONE',  ( -4.499999999999999112, -0.5000000000000009992, -65.00000000000000000 ) ) ;
#7580=ORIENTED_EDGE ( 'NONE', *, *, #12866, .F. ) ;
#7581=DIRECTION ( 'NONE',  ( -1.000000000000000000, -2.529805069132845816E-16, -0.000000000000000000 ) ) ;
#7679=ORIENTED_EDGE ( 'NONE', *, *, #544, .T. ) ;
#7702=DIRECTION ( 'NONE',  ( -1.000000000000000000, -1.239088197126292296E-16, -0.000000000000000000 ) ) ;
#7705=LINE ( 'NONE', #3412, #6936 ) ;
#7792=LINE ( 'NONE', #10189, #2048 ) ;
#7845=ORIENTED_EDGE ( 'NONE', *, *, #5887, .T. ) ;
#7851=LINE ( 'NONE', #2511, #5321 ) ;
#7932=ADVANCED_FACE ( 'NONE', ( #3082 ), #4956, .T. ) ;
#7933=FACE_OUTER_BOUND ( 'NONE', #11598, .T. ) ;
#7994=CARTESIAN_POINT ( 'NONE',  ( -8.499999999999998224, 2.000000000000000000, -65.00000000000000000 ) ) ;
#7995=DIRECTION ( 'NONE',  ( 3.614007241618347908E-17, -1.000000000000000000, 0.000000000000000000 ) ) ;
#8009=DIRECTION ( 'NONE',  ( 1.000000000000000000, 3.614007241618347908E-17, 0.000000000000000000 ) ) ;
#8021=AXIS2_PLACEMENT_3D ( 'NONE', #11185, #4697, #1613 ) ;
#8044=AXIS2_PLACEMENT_3D ( 'NONE', #13728, #8221, #8362 ) ;
#8071=DIRECTION ( 'NONE',  ( 1.000000000000000000, 0.000000000000000000, -0.000000000000000000 ) ) ;
#8088=DIRECTION ( 'NONE',  ( 0.000000000000000000, 0.000000000000000000, 1.000000000000000000 ) ) ;
#8099=ORIENTED_EDGE ( 'NONE', *, *, #3948, .T. ) ;
#8133=CARTESIAN_POINT ( 'NONE',  ( -8.499999999999998224, 2.000000000000000000, -65.00000000000000000 ) ) ;
#8144=CARTESIAN_POINT ( 'NONE',  ( -7.999999999999998224, 2.000000000000000000, -65.00000000000000000 ) ) ;
#8162=VERTEX_POINT ( 'NONE', #3753 ) ;
#8167=EDGE_CURVE ( 'NONE', #3998, #11468, #8992, .T. ) ;
#8173=ORIENTED_EDGE ( 'NONE', *, *, #3970, .T. ) ;
#8202=CIRCLE ( 'NONE', #8421, 0.5000000000000000000 ) ;
#8221=DIRECTION ( 'NONE',  ( 0.000000000000000000, 0.000000000000000000, 1.000000000000000000 ) ) ;
#8231=ORIENTED_EDGE ( 'NONE', *, *, #13794, .T. ) ;
#8241=ADVANCED_FACE ( 'NONE', ( #1303 ), #10885, .T. ) ;
#8362=DIRECTION ( 'NONE',  ( 1.000000000000000000, 0.000000000000000000, 0.000000000000000000 ) ) ;
#8380=DIRECTION ( 'NONE',  ( 1.000000000000000000, 0.000000000000000000, 0.000000000000000000 ) ) ;
#8384=VERTEX_POINT ( 'NONE', #1796 ) ;
#8421=AXIS2_PLACEMENT_3D ( 'NONE', #169, #3407, #4446 ) ;
#8454=CARTESIAN_POINT ( 'NONE',  ( -8.500000000000000000, 2.499999999999999556, 0.000000000000000000 ) ) ;
#8472=DIRECTION ( 'NONE',  ( 1.000000000000000000, 0.000000000000000000, 0.000000000000000000 ) ) ;
#8484=LINE ( 'NONE', #2151, #6602 ) ;
#8492=CIRCLE ( 'NONE', #4273, 0.5000000000000004441 ) ;
#8507=ORIENTED_EDGE ( 'NONE', *, *, #414, .F. ) ;
#8510=DIRECTION ( 'NONE',  ( 5.059610138265691632E-16, 1.000000000000000000, -0.000000000000000000 ) ) ;
#8514=DIRECTION ( 'NONE',  ( 0.000000000000000000, 0.000000000000000000, 1.000000000000000000 ) ) ;
#8521=VERTEX_POINT ( 'NONE', #13718 ) ;
#8561=LINE ( 'NONE', #3276, #3350 ) ;
#8562=EDGE_CURVE ( 'NONE', #8521, #9884, #8484, .T. ) ;
#8578=ADVANCED_FACE ( 'NONE', ( #9953 ), #4723, .T. ) ;
#8585=AXIS2_PLACEMENT_3D ( 'NONE', #9222, #3977, #7298 ) ;
#8589=DIRECTION ( 'NONE',  ( -1.000000000000000000, 5.059610138265691632E-16, 0.000000000000000000 ) ) ;
#8591=DIRECTION ( 'NONE',  ( -1.000000000000000000, -0.000000000000000000, -0.000000000000000000 ) ) ;
#8604=DIRECTION ( 'NONE',  ( -1.000000000000000000, 0.000000000000000000, 0.000000000000000000 ) ) ;
#8629=SHAPE_REPRESENTATION_RELATIONSHIP ( 'NONE' , 'NONE' ,  #5502, #9430 ) ;
#8652=VECTOR ( 'NONE', #12590, 1000.000000000000000 ) ;
#8673=EDGE_CURVE ( 'NONE', #11152, #6401, #378, .T. ) ;
#8676=PRODUCT_DEFINITION_FORMATION_WITH_SPECIFIED_SOURCE ( 'ANY', '', #5400, .NOT_KNOWN. ) ;
#8681=CARTESIAN_POINT ( 'NONE',  ( -7.499999999999996447, -0.5000000000000019984, -65.00000000000000000 ) ) ;
#8767=EDGE_CURVE ( 'NONE', #2349, #4357, #5888, .T. ) ;
#8787=CARTESIAN_POINT ( 'NONE',  ( -7.499999999999996447, -0.5000000000000017764, -65.00000000000000000 ) ) ;
#8789=DIRECTION ( 'NONE',  ( 0.000000000000000000, 0.000000000000000000, 1.000000000000000000 ) ) ;
#8807=DIRECTION ( 'NONE',  ( -8.673617379884027583E-16, -1.000000000000000000, 0.000000000000000000 ) ) ;
#8834=FACE_OUTER_BOUND ( 'NONE', #10969, .T. ) ;
#8845=APPLICATION_CONTEXT ( 'automotive_design' ) ;
#8847=ORIENTED_EDGE ( 'NONE', *, *, #1648, .T. ) ;
#8884=AXIS2_PLACEMENT_3D ( 'NONE', #11481, #10305, #4990 ) ;
#8888=VERTEX_POINT ( 'NONE', #5302 ) ;
#8910=DIRECTION ( 'NONE',  ( -0.000000000000000000, -0.000000000000000000, -1.000000000000000000 ) ) ;
#8931=CARTESIAN_POINT ( 'NONE',  ( -3.999999999999997335, 2.000000000000000000, -65.00000000000000000 ) ) ;
#8954=AXIS2_PLACEMENT_3D ( 'NONE', #7009, #7995, #4658 ) ;
#8992=LINE ( 'NONE', #6815, #9280 ) ;
#9005=CARTESIAN_POINT ( 'NONE',  ( 4.000000000000001776, -4.336808689942017736E-16, -65.00000000000000000 ) ) ;
#9009=EDGE_LOOP ( 'NONE', ( #10137, #9589, #3591, #7845 ) ) ;
#9021=ORIENTED_EDGE ( 'NONE', *, *, #9638, .F. ) ;
#9022=ORIENTED_EDGE ( 'NONE', *, *, #4814, .T. ) ;
#9052=DIRECTION ( 'NONE',  ( 0.000000000000000000, 0.000000000000000000, 1.000000000000000000 ) ) ;
#9059=CARTESIAN_POINT ( 'NONE',  ( 8.500000000000003553, 2.499999999999999556, -65.00000000000000000 ) ) ;
#9116=DIRECTION ( 'NONE',  ( 1.000000000000000000, 0.000000000000000000, 0.000000000000000000 ) ) ;
#9120=PRODUCT_CONTEXT ( 'NONE', #9304, 'mechanical' ) ;
#9132=ADVANCED_FACE ( 'NONE', ( #11451 ), #10545, .F. ) ;
#9144=VERTEX_POINT ( 'NONE', #13536 ) ;
#9170=PLANE ( 'NONE',  #905 ) ;
#9190=CARTESIAN_POINT ( 'NONE',  ( 7.500000000000000000, -0.5000000000000017764, 0.000000000000000000 ) ) ;
#9193=FACE_OUTER_BOUND ( 'NONE', #1493, .T. ) ;
#9222=CARTESIAN_POINT ( 'NONE',  ( -7.999999999999998224, 2.000000000000000000, -65.00000000000000000 ) ) ;
#9235=ORIENTED_EDGE ( 'NONE', *, *, #9892, .F. ) ;
#9250=EDGE_CURVE ( 'NONE', #2367, #5154, #10751, .T. ) ;
#9268=ORIENTED_EDGE ( 'NONE', *, *, #1917, .T. ) ;
#9272=CARTESIAN_POINT ( 'NONE',  ( -7.999999999999998224, 2.000000000000000000, -65.00000000000000000 ) ) ;
#9275=DIRECTION ( 'NONE',  ( 1.000000000000000000, 0.000000000000000000, 0.000000000000000000 ) ) ;
#9280=VECTOR ( 'NONE', #5836, 1000.000000000000000 ) ;
#9284=ORIENTED_EDGE ( 'NONE', *, *, #1407, .T. ) ;
#9304=APPLICATION_CONTEXT ( 'automotive_design' ) ;
#9307=DIRECTION ( 'NONE',  ( 1.000000000000000000, 0.000000000000000000, 0.000000000000000000 ) ) ;
#9321=AXIS2_PLACEMENT_3D ( 'NONE', #8133, #2852, #6524 ) ;
#9345=AXIS2_PLACEMENT_3D ( 'NONE', #3697, #3843, #6768 ) ;
#9362=CIRCLE ( 'NONE', #2018, 0.5000000000000004441 ) ;
#9391=VECTOR ( 'NONE', #13786, 1000.000000000000000 ) ;
#9401=FACE_OUTER_BOUND ( 'NONE', #11951, .T. ) ;
#9407=ORIENTED_EDGE ( 'NONE', *, *, #4860, .T. ) ;
#9411=EDGE_CURVE ( 'NONE', #2347, #6401, #401, .T. ) ;
#9430=ADVANCED_BREP_SHAPE_REPRESENTATION ( '', ( #4577, #6434 ), #1075 ) ;
#9469=EDGE_CURVE ( 'NONE', #10379, #1230, #12480, .T. ) ;
#9530=ORIENTED_EDGE ( 'NONE', *, *, #12612, .T. ) ;
#9563=AXIS2_PLACEMENT_3D ( 'NONE', #992, #1983, #9307 ) ;
#9581=VECTOR ( 'NONE', #2497, 1000.000000000000000 ) ;
#9589=ORIENTED_EDGE ( 'NONE', *, *, #8562, .F. ) ;
#9611=DIRECTION ( 'NONE',  ( -1.000000000000000000, 0.000000000000000000, 0.000000000000000000 ) ) ;
#9619=EDGE_LOOP ( 'NONE', ( #11658, #7580, #10865, #1245 ) ) ;
#9638=EDGE_CURVE ( 'NONE', #12422, #2347, #8202, .T. ) ;
#9640=DIRECTION ( 'NONE',  ( 1.000000000000000000, 0.000000000000000000, 0.000000000000000000 ) ) ;
#9659=CIRCLE ( 'NONE', #7396, 0.5000000000000004441 ) ;
#9662=ORIENTED_EDGE ( 'NONE', *, *, #5380, .T. ) ;
#9684=DIRECTION ( 'NONE',  ( 0.000000000000000000, 0.000000000000000000, 1.000000000000000000 ) ) ;
#9692=CARTESIAN_POINT ( 'NONE',  ( -3.999999999999997335, 2.000000000000000000, -65.00000000000000000 ) ) ;
#9703=ORIENTED_EDGE ( 'NONE', *, *, #1167, .F. ) ;
#9716=CARTESIAN_POINT ( 'NONE',  ( -12.00000000000000000, 2.500000000000000000, -65.00000000000000000 ) ) ;
#9740=ORIENTED_EDGE ( 'NONE', *, *, #2965, .F. ) ;
#9757=ORIENTED_EDGE ( 'NONE', *, *, #3592, .F. ) ;
#9822=CIRCLE ( 'NONE', #10703, 0.5000000000000000000 ) ;
#9833=CARTESIAN_POINT ( 'NONE',  ( -7.499999999999996447, -0.5000000000000019984, -65.00000000000000000 ) ) ;
#9855=CARTESIAN_POINT ( 'NONE',  ( 12.00000000000000000, -2.499999999999999556, -65.00000000000000000 ) ) ;
#9878=EDGE_LOOP ( 'NONE', ( #685, #4082, #6423, #6811 ) ) ;
#9884=VERTEX_POINT ( 'NONE', #654 ) ;
#9892=EDGE_CURVE ( 'NONE', #2367, #11937, #11349, .T. ) ;
#9926=ORIENTED_EDGE ( 'NONE', *, *, #80, .T. ) ;
#9932=PLANE ( 'NONE',  #12713 ) ;
#9933=EDGE_CURVE ( 'NONE', #11152, #4755, #3099, .T. ) ;
#9953=FACE_OUTER_BOUND ( 'NONE', #4188, .T. ) ;
#9982=CARTESIAN_POINT ( 'NONE',  ( 4.000000000000001776, 2.000000000000000000, 0.000000000000000000 ) ) ;
#10033=VECTOR ( 'NONE', #294, 1000.000000000000000 ) ;
#10060=PLANE ( 'NONE',  #12061 ) ;
#10061=PRODUCT_DEFINITION ( 'UNKNOWN', '', #8676, #12566 ) ;
#10066=AXIS2_PLACEMENT_3D ( 'NONE', #13115, #6618, #10893 ) ;
#10075=CARTESIAN_POINT ( 'NONE',  ( -4.499999999999999112, -0.5000000000000009992, 0.000000000000000000 ) ) ;
#10092=ORIENTED_EDGE ( 'NONE', *, *, #13036, .F. ) ;
#10097=CARTESIAN_POINT ( 'NONE',  ( 8.000000000000001776, 2.000000000000000000, 0.000000000000000000 ) ) ;
#10101=MECHANICAL_DESIGN_GEOMETRIC_PRESENTATION_REPRESENTATION('',(#5381),#37);
#10130=FACE_OUTER_BOUND ( 'NONE', #5449, .T. ) ;
#10134=VECTOR ( 'NONE', #12151, 1000.000000000000000 ) ;
#10137=ORIENTED_EDGE ( 'NONE', *, *, #13794, .F. ) ;
#10177=CARTESIAN_POINT ( 'NONE',  ( 7.500000000000000000, -1.762812401309176307E-15, -65.00000000000000000 ) ) ;
#10189=CARTESIAN_POINT ( 'NONE',  ( -12.00000000000000000, -2.500000000000000444, -65.00000000000000000 ) ) ;
#10194=VECTOR ( 'NONE', #5742, 1000.000000000000000 ) ;
#10269=AXIS2_PLACEMENT_3D ( 'NONE', #10177, #2854, #7212 ) ;
#10292=EDGE_LOOP ( 'NONE', ( #3516, #1259, #391, #1476 ) ) ;
#10303=VERTEX_POINT ( 'NONE', #13350 ) ;
#10305=DIRECTION ( 'NONE',  ( 0.000000000000000000, 0.000000000000000000, 1.000000000000000000 ) ) ;
#10314=EDGE_LOOP ( 'NONE', ( #3216, #7172, #1719, #7679 ) ) ;
#10326=CARTESIAN_POINT ( 'NONE',  ( -4.499999999999999112, -1.301042606982605321E-15, 0.000000000000000000 ) ) ;
#10351=CARTESIAN_POINT ( 'NONE',  ( -12.00000000000000000, 2.500000000000000000, -65.00000000000000000 ) ) ;
#10379=VERTEX_POINT ( 'NONE', #10418 ) ;
#10394=ORIENTED_EDGE ( 'NONE', *, *, #11857, .F. ) ;
#10418=CARTESIAN_POINT ( 'NONE',  ( -7.999999999999996447, -1.701580061351808733E-15, -65.00000000000000000 ) ) ;
#10460=DIRECTION ( 'NONE',  ( 1.000000000000000000, 0.000000000000000000, 0.000000000000000000 ) ) ;
#10543=ORIENTED_EDGE ( 'NONE', *, *, #11857, .T. ) ;
#10545=CYLINDRICAL_SURFACE ( 'NONE', #11309, 0.5000000000000004441 ) ;
#10562=FACE_OUTER_BOUND ( 'NONE', #6353, .T. ) ;
#10572=VERTEX_POINT ( 'NONE', #12148 ) ;
#10589=CARTESIAN_POINT ( 'NONE',  ( 8.500000000000003553, 2.500000000000000000, -65.00000000000000000 ) ) ;
#10613=CARTESIAN_POINT ( 'NONE',  ( 12.00000000000000000, -2.499999999999999556, -65.00000000000000000 ) ) ;
#10642=ORIENTED_EDGE ( 'NONE', *, *, #926, .T. ) ;
#10644=CARTESIAN_POINT ( 'NONE',  ( 8.500000000000001776, 2.000000000000000000, -65.00000000000000000 ) ) ;
#10651=DIRECTION ( 'NONE',  ( 0.000000000000000000, 0.000000000000000000, 1.000000000000000000 ) ) ;
#10654=CARTESIAN_POINT ( 'NONE',  ( 8.500000000000001776, 2.000000000000000000, 0.000000000000000000 ) ) ;
#10663=CARTESIAN_POINT ( 'NONE',  ( 4.000000000000001776, -4.336808689942017736E-16, -65.00000000000000000 ) ) ;
#10679=CARTESIAN_POINT ( 'NONE',  ( 12.00000000000000000, -2.499999999999999556, 0.000000000000000000 ) ) ;
#10685=DIRECTION ( 'NONE',  ( 0.000000000000000000, 0.000000000000000000, 1.000000000000000000 ) ) ;
#10699=CARTESIAN_POINT ( 'NONE',  ( -3.499999999999998224, 2.499999999999999556, -65.00000000000000000 ) ) ;
#10703=AXIS2_PLACEMENT_3D ( 'NONE', #870, #797, #12270 ) ;
#10728=DIRECTION ( 'NONE',  ( 0.000000000000000000, 0.000000000000000000, 1.000000000000000000 ) ) ;
#10751=LINE ( 'NONE', #8787, #3517 ) ;
#10752=CARTESIAN_POINT ( 'NONE',  ( -8.499999999999998224, 2.000000000000000000, -65.00000000000000000 ) ) ;
#10813=VERTEX_POINT ( 'NONE', #5412 ) ;
#10819=CYLINDRICAL_SURFACE ( 'NONE', #1815, 0.5000000000000004441 ) ;
#10834=LINE ( 'NONE', #11949, #7138 ) ;
#10852=CARTESIAN_POINT ( 'NONE',  ( -7.499999999999996447, -1.762812401309176307E-15, -65.00000000000000000 ) ) ;
#10865=ORIENTED_EDGE ( 'NONE', *, *, #3131, .T. ) ;
#10879=( LENGTH_UNIT ( ) NAMED_UNIT ( * ) SI_UNIT ( .MILLI., .METRE. ) );
#10885=PLANE ( 'NONE',  #1919 ) ;
#10893=DIRECTION ( 'NONE',  ( 1.000000000000000000, 0.000000000000000000, 0.000000000000000000 ) ) ;
#10909=ORIENTED_EDGE ( 'NONE', *, *, #12866, .T. ) ;
#10929=LINE ( 'NONE', #10097, #2065 ) ;
#10940=AXIS2_PLACEMENT_3D ( 'NONE', #11258, #627, #11320 ) ;
#10949=CARTESIAN_POINT ( 'NONE',  ( 8.500000000000003553, 2.499999999999999556, 0.000000000000000000 ) ) ;
#10955=CIRCLE ( 'NONE', #4919, 0.4999999999999991673 ) ;
#10965=CARTESIAN_POINT ( 'NONE',  ( -7.499999999999996447, -0.5000000000000017764, -65.00000000000000000 ) ) ;
#10969=EDGE_LOOP ( 'NONE', ( #1900, #5870, #6499, #1620 ) ) ;
#10975=DIRECTION ( 'NONE',  ( 0.000000000000000000, 1.000000000000000000, 0.000000000000000000 ) ) ;
#10990=EDGE_CURVE ( 'NONE', #10379, #3647, #7851, .T. ) ;
#11012=ORIENTED_EDGE ( 'NONE', *, *, #161, .F. ) ;
#11064=ORIENTED_EDGE ( 'NONE', *, *, #3455, .F. ) ;
#11071=ADVANCED_FACE ( 'NONE', ( #7933 ), #4673, .T. ) ;
#11081=CARTESIAN_POINT ( 'NONE',  ( 3.500000000000001776, 2.499999999999999556, -65.00000000000000000 ) ) ;
#11086=ADVANCED_FACE ( 'NONE', ( #5635 ), #5768, .T. ) ;
#11122=VECTOR ( 'NONE', #12602, 1000.000000000000000 ) ;
#11152=VERTEX_POINT ( 'NONE', #2389 ) ;
#11164=ADVANCED_FACE ( 'NONE', ( #4537 ), #5563, .T. ) ;
#11185=CARTESIAN_POINT ( 'NONE',  ( -8.499999999999998224, 2.000000000000000000, 0.000000000000000000 ) ) ;
#11216=DIRECTION ( 'NONE',  ( 0.000000000000000000, 0.000000000000000000, 1.000000000000000000 ) ) ;
#11222=FACE_OUTER_BOUND ( 'NONE', #12426, .T. ) ;
#11255=SURFACE_STYLE_USAGE ( .BOTH. , #825 ) ;
#11258=CARTESIAN_POINT ( 'NONE',  ( -7.499999999999996447, -1.762812401309176307E-15, 0.000000000000000000 ) ) ;
#11277=ORIENTED_EDGE ( 'NONE', *, *, #13036, .T. ) ;
#11284=CARTESIAN_POINT ( 'NONE',  ( 8.000000000000000000, -1.762812401309176307E-15, -65.00000000000000000 ) ) ;
#11292=ORIENTED_EDGE ( 'NONE', *, *, #6474, .F. ) ;
#11309=AXIS2_PLACEMENT_3D ( 'NONE', #6281, #1823, #687 ) ;
#11320=DIRECTION ( 'NONE',  ( -1.000000000000000000, 0.000000000000000000, 0.000000000000000000 ) ) ;
#11349=LINE ( 'NONE', #7145, #11122 ) ;
#11350=EDGE_CURVE ( 'NONE', #5154, #10379, #5079, .T. ) ;
#11356=CARTESIAN_POINT ( 'NONE',  ( -12.00000000000000000, 2.500000000000000000, -65.00000000000000000 ) ) ;
#11401=VECTOR ( 'NONE', #901, 1000.000000000000000 ) ;
#11411=VECTOR ( 'NONE', #13709, 1000.000000000000000 ) ;
#11451=FACE_OUTER_BOUND ( 'NONE', #9009, .T. ) ;
#11468=VERTEX_POINT ( 'NONE', #2205 ) ;
#11477=ORIENTED_EDGE ( 'NONE', *, *, #12293, .T. ) ;
#11481=CARTESIAN_POINT ( 'NONE',  ( -3.499999999999998224, 2.000000000000000000, -65.00000000000000000 ) ) ;
#11507=DIRECTION ( 'NONE',  ( -0.000000000000000000, -0.000000000000000000, -1.000000000000000000 ) ) ;
#11508=ORIENTED_EDGE ( 'NONE', *, *, #4814, .F. ) ;
#11510=ORIENTED_EDGE ( 'NONE', *, *, #5344, .F. ) ;
#11521=DIRECTION ( 'NONE',  ( 0.000000000000000000, 0.000000000000000000, 1.000000000000000000 ) ) ;
#11527=ORIENTED_EDGE ( 'NONE', *, *, #5186, .F. ) ;
#11544=VERTEX_POINT ( 'NONE', #3664 ) ;
#11598=EDGE_LOOP ( 'NONE', ( #4103, #6157, #4088, #11477 ) ) ;
#11651=DIRECTION ( 'NONE',  ( -0.000000000000000000, 1.000000000000000000, -0.000000000000000000 ) ) ;
#11654=CARTESIAN_POINT ( 'NONE',  ( 0.000000000000000000, 0.000000000000000000, 0.000000000000000000 ) ) ;
#11655=ADVANCED_FACE ( 'NONE', ( #10562 ), #2904, .F. ) ;
#11656=EDGE_CURVE ( 'NONE', #2349, #2553, #6078, .T. ) ;
#11658=ORIENTED_EDGE ( 'NONE', *, *, #9411, .F. ) ;
#11709=CARTESIAN_POINT ( 'NONE',  ( -3.499999999999998224, 2.000000000000000000, 0.000000000000000000 ) ) ;
#11714=LINE ( 'NONE', #3142, #2462 ) ;
#11724=DIRECTION ( 'NONE',  ( 0.000000000000000000, 0.000000000000000000, 1.000000000000000000 ) ) ;
#11798=VECTOR ( 'NONE', #8807, 1000.000000000000000 ) ;
#11807=ORIENTED_EDGE ( 'NONE', *, *, #9469, .F. ) ;
#11826=DIRECTION ( 'NONE',  ( -0.000000000000000000, -0.000000000000000000, -1.000000000000000000 ) ) ;
#11837=VECTOR ( 'NONE', #5107, 1000.000000000000000 ) ;
#11856=DIRECTION ( 'NONE',  ( 1.000000000000000000, 0.000000000000000000, 0.000000000000000000 ) ) ;
#11857=EDGE_CURVE ( 'NONE', #10813, #8521, #4349, .T. ) ;
#11903=CARTESIAN_POINT ( 'NONE',  ( -3.999999999999997335, 2.000000000000000000, 0.000000000000000000 ) ) ;
#11913=DIRECTION ( 'NONE',  ( -8.673617379884027583E-16, -1.000000000000000000, 0.000000000000000000 ) ) ;
#11937=VERTEX_POINT ( 'NONE', #10075 ) ;
#11949=CARTESIAN_POINT ( 'NONE',  ( 7.500000000000000000, -0.5000000000000017764, -65.00000000000000000 ) ) ;
#11951=EDGE_LOOP ( 'NONE', ( #2540, #12925, #1658, #5204, #5384, #6444, #11807, #12300, #1999, #5871, #2848, #1077, #4686, #11292, #3464, #366, #10394, #6394, #2239, #317 ) ) ;
#11963=VERTEX_POINT ( 'NONE', #426 ) ;
#11966=ORIENTED_EDGE ( 'NONE', *, *, #9469, .T. ) ;
#12023=CARTESIAN_POINT ( 'NONE',  ( 4.000000000000001776, 2.000000000000000000, -65.00000000000000000 ) ) ;
#12050=ORIENTED_EDGE ( 'NONE', *, *, #3970, .F. ) ;
#12053=DIRECTION ( 'NONE',  ( 1.000000000000000000, 0.000000000000000000, 0.000000000000000000 ) ) ;
#12061=AXIS2_PLACEMENT_3D ( 'NONE', #9059, #408, #13318 ) ;
#12063=AXIS2_PLACEMENT_3D ( 'NONE', #1385, #8510, #1098 ) ;
#12069=CARTESIAN_POINT ( 'NONE',  ( -3.499999999999998224, 2.499999999999999556, 0.000000000000000000 ) ) ;
#12095=LINE ( 'NONE', #4556, #10033 ) ;
#12101=EDGE_LOOP ( 'NONE', ( #3417, #1258, #11966, #9022 ) ) ;
#12115=CARTESIAN_POINT ( 'NONE',  ( 4.000000000000001776, 2.000000000000000000, 0.000000000000000000 ) ) ;
#12134=ORIENTED_EDGE ( 'NONE', *, *, #11350, .T. ) ;
#12146=CARTESIAN_POINT ( 'NONE',  ( -7.999999999999998224, 2.000000000000000000, -65.00000000000000000 ) ) ;
#12148=CARTESIAN_POINT ( 'NONE',  ( 8.000000000000000000, -1.762812401309176307E-15, 0.000000000000000000 ) ) ;
#12151=DIRECTION ( 'NONE',  ( 0.000000000000000000, 0.000000000000000000, 1.000000000000000000 ) ) ;
#12193=DIRECTION ( 'NONE',  ( 0.000000000000000000, 0.000000000000000000, 1.000000000000000000 ) ) ;
#12207=CARTESIAN_POINT ( 'NONE',  ( -3.499999999999998224, 2.499999999999999556, -65.00000000000000000 ) ) ;
#12226=AXIS2_PLACEMENT_3D ( 'NONE', #9855, #13045, #6760 ) ;
#12270=DIRECTION ( 'NONE',  ( 1.000000000000000000, 0.000000000000000000, 0.000000000000000000 ) ) ;
#12293=EDGE_CURVE ( 'NONE', #8888, #5295, #6411, .T. ) ;
#12300=ORIENTED_EDGE ( 'NONE', *, *, #11350, .F. ) ;
#12355=CARTESIAN_POINT ( 'NONE',  ( 4.500000000000002665, -4.336808689942017736E-16, -65.00000000000000000 ) ) ;
#12382=ORIENTED_EDGE ( 'NONE', *, *, #9933, .T. ) ;
#12422=VERTEX_POINT ( 'NONE', #9982 ) ;
#12426=EDGE_LOOP ( 'NONE', ( #9703, #11510, #9268, #13626 ) ) ;
#12465=ORIENTED_EDGE ( 'NONE', *, *, #12551, .F. ) ;
#12469=CARTESIAN_POINT ( 'NONE',  ( -7.499999999999996447, -0.5000000000000017764, 0.000000000000000000 ) ) ;
#12480=LINE ( 'NONE', #8144, #12861 ) ;
#12551=EDGE_CURVE ( 'NONE', #2380, #12422, #1660, .T. ) ;
#12566=PRODUCT_DEFINITION_CONTEXT ( 'detailed design', #8845, 'design' ) ;
#12572=ORIENTED_EDGE ( 'NONE', *, *, #490, .F. ) ;
#12574=DIRECTION ( 'NONE',  ( -0.000000000000000000, -1.000000000000000000, -0.000000000000000000 ) ) ;
#12581=ORIENTED_EDGE ( 'NONE', *, *, #9411, .T. ) ;
#12585=CARTESIAN_POINT ( 'NONE',  ( -8.500000000000000000, 2.499999999999999556, -65.00000000000000000 ) ) ;
#12590=DIRECTION ( 'NONE',  ( -1.000000000000000000, 1.239088197126291063E-16, -0.000000000000000000 ) ) ;
#12602=DIRECTION ( 'NONE',  ( 0.000000000000000000, 0.000000000000000000, 1.000000000000000000 ) ) ;
#12612=EDGE_CURVE ( 'NONE', #5295, #11937, #646, .T. ) ;
#12699=VECTOR ( 'NONE', #8589, 1000.000000000000000 ) ;
#12713=AXIS2_PLACEMENT_3D ( 'NONE', #12023, #4762, #4554 ) ;
#12736=AXIS2_PLACEMENT_3D ( 'NONE', #12355, #339, #13187 ) ;
#12753=EDGE_CURVE ( 'NONE', #2257, #2380, #11714, .T. ) ;
#12754=ORIENTED_EDGE ( 'NONE', *, *, #80, .F. ) ;
#12766=CIRCLE ( 'NONE', #4301, 0.5000000000000004441 ) ;
#12825=DIRECTION ( 'NONE',  ( 0.000000000000000000, 0.000000000000000000, 1.000000000000000000 ) ) ;
#12861=VECTOR ( 'NONE', #7088, 1000.000000000000000 ) ;
#12866=EDGE_CURVE ( 'NONE', #11544, #2347, #13170, .T. ) ;
#12925=ORIENTED_EDGE ( 'NONE', *, *, #2306, .F. ) ;
#12947=VECTOR ( 'NONE', #10975, 1000.000000000000000 ) ;
#12953=CARTESIAN_POINT ( 'NONE',  ( 8.000000000000001776, 2.000000000000000000, -65.00000000000000000 ) ) ;
#12974=CARTESIAN_POINT ( 'NONE',  ( -7.999999999999996447, -1.701580061351808733E-15, 0.000000000000000000 ) ) ;
#12978=DIRECTION ( 'NONE',  ( 0.000000000000000000, 0.000000000000000000, 1.000000000000000000 ) ) ;
#12993=EDGE_CURVE ( 'NONE', #3627, #10303, #2718, .T. ) ;
#12999=CARTESIAN_POINT ( 'NONE',  ( 8.000000000000001776, 2.000000000000000000, -65.00000000000000000 ) ) ;
#13000=AXIS2_PLACEMENT_3D ( 'NONE', #1859, #13443, #9116 ) ;
#13014=ADVANCED_FACE ( 'NONE', ( #9401 ), #3744, .F. ) ;
#13028=CARTESIAN_POINT ( 'NONE',  ( -4.499999999999999112, -1.301042606982605321E-15, -65.00000000000000000 ) ) ;
#13036=EDGE_CURVE ( 'NONE', #11937, #11963, #657, .T. ) ;
#13045=DIRECTION ( 'NONE',  ( 1.000000000000000000, 0.000000000000000000, 0.000000000000000000 ) ) ;
#13047=LINE ( 'NONE', #12146, #4289 ) ;
#13050=ADVANCED_FACE ( 'NONE', ( #9193 ), #3888, .T. ) ;
#13069=ORIENTED_EDGE ( 'NONE', *, *, #1167, .T. ) ;
#13089=DIRECTION ( 'NONE',  ( -1.000000000000000000, 8.673617379884027583E-16, 0.000000000000000000 ) ) ;
#13095=LINE ( 'NONE', #10949, #6964 ) ;
#13115=CARTESIAN_POINT ( 'NONE',  ( 7.500000000000000000, -1.762812401309176307E-15, -65.00000000000000000 ) ) ;
#13165=ORIENTED_EDGE ( 'NONE', *, *, #3592, .T. ) ;
#13170=LINE ( 'NONE', #11081, #6208 ) ;
#13187=DIRECTION ( 'NONE',  ( 1.000000000000000000, 0.000000000000000000, 0.000000000000000000 ) ) ;
#13236=CARTESIAN_POINT ( 'NONE',  ( -3.499999999999998224, 2.499999999999999556, -65.00000000000000000 ) ) ;
#13318=DIRECTION ( 'NONE',  ( -1.000000000000000000, -1.239088197126292296E-16, 0.000000000000000000 ) ) ;
#13321=FACE_OUTER_BOUND ( 'NONE', #1649, .T. ) ;
#13350=CARTESIAN_POINT ( 'NONE',  ( 12.00000000000000000, -2.499999999999999556, 0.000000000000000000 ) ) ;
#13356=LINE ( 'NONE', #12115, #9581 ) ;
#13376=ADVANCED_FACE ( 'NONE', ( #694 ), #3031, .T. ) ;
#13409=FILL_AREA_STYLE ('',( #6199 ) ) ;
#13424=DIRECTION ( 'NONE',  ( 1.239088197126291063E-16, 1.000000000000000000, -0.000000000000000000 ) ) ;
#13443=DIRECTION ( 'NONE',  ( 0.000000000000000000, 0.000000000000000000, 1.000000000000000000 ) ) ;
#13503=LINE ( 'NONE', #9190, #11411 ) ;
#13516=ORIENTED_EDGE ( 'NONE', *, *, #9250, .T. ) ;
#13534=EDGE_LOOP ( 'NONE', ( #5940, #12572, #10543, #6009 ) ) ;
#13536=CARTESIAN_POINT ( 'NONE',  ( 8.000000000000001776, 2.000000000000000000, -65.00000000000000000 ) ) ;
#13538=CARTESIAN_POINT ( 'NONE',  ( -3.999999999999997335, 2.000000000000000000, -65.00000000000000000 ) ) ;
#13543=VECTOR ( 'NONE', #4672, 1000.000000000000000 ) ;
#13544=EDGE_CURVE ( 'NONE', #4291, #10303, #7439, .T. ) ;
#13553=CARTESIAN_POINT ( 'NONE',  ( 12.00000000000000000, 2.500000000000000000, -65.00000000000000000 ) ) ;
#13584=VERTEX_POINT ( 'NONE', #5848 ) ;
#13606=ORIENTED_EDGE ( 'NONE', *, *, #8767, .T. ) ;
#13615=AXIS2_PLACEMENT_3D ( 'NONE', #3687, #9052, #3754 ) ;
#13626=ORIENTED_EDGE ( 'NONE', *, *, #490, .T. ) ;
#13657=ADVANCED_FACE ( 'NONE', ( #13321 ), #5642, .T. ) ;
#13667=VERTEX_POINT ( 'NONE', #2741 ) ;
#13676=ORIENTED_EDGE ( 'NONE', *, *, #2965, .T. ) ;
#13709=DIRECTION ( 'NONE',  ( -1.000000000000000000, 5.059610138265691632E-16, 0.000000000000000000 ) ) ;
#13718=CARTESIAN_POINT ( 'NONE',  ( 4.500000000000002665, -0.5000000000000005551, -65.00000000000000000 ) ) ;
#13728=CARTESIAN_POINT ( 'NONE',  ( 3.500000000000001776, 2.000000000000000000, -65.00000000000000000 ) ) ;
#13752=VECTOR ( 'NONE', #98, 1000.000000000000000 ) ;
#13770=DIRECTION ( 'NONE',  ( 0.000000000000000000, 0.000000000000000000, 1.000000000000000000 ) ) ;
#13786=DIRECTION ( 'NONE',  ( -0.000000000000000000, -1.000000000000000000, -0.000000000000000000 ) ) ;
#13794=EDGE_CURVE ( 'NONE', #9884, #13584, #5758, .T. ) ;
#13795=DIRECTION ( 'NONE',  ( -1.000000000000000000, 1.239088197126291063E-16, -0.000000000000000000 ) ) ;
ENDSEC;
END-ISO-10303-21;
